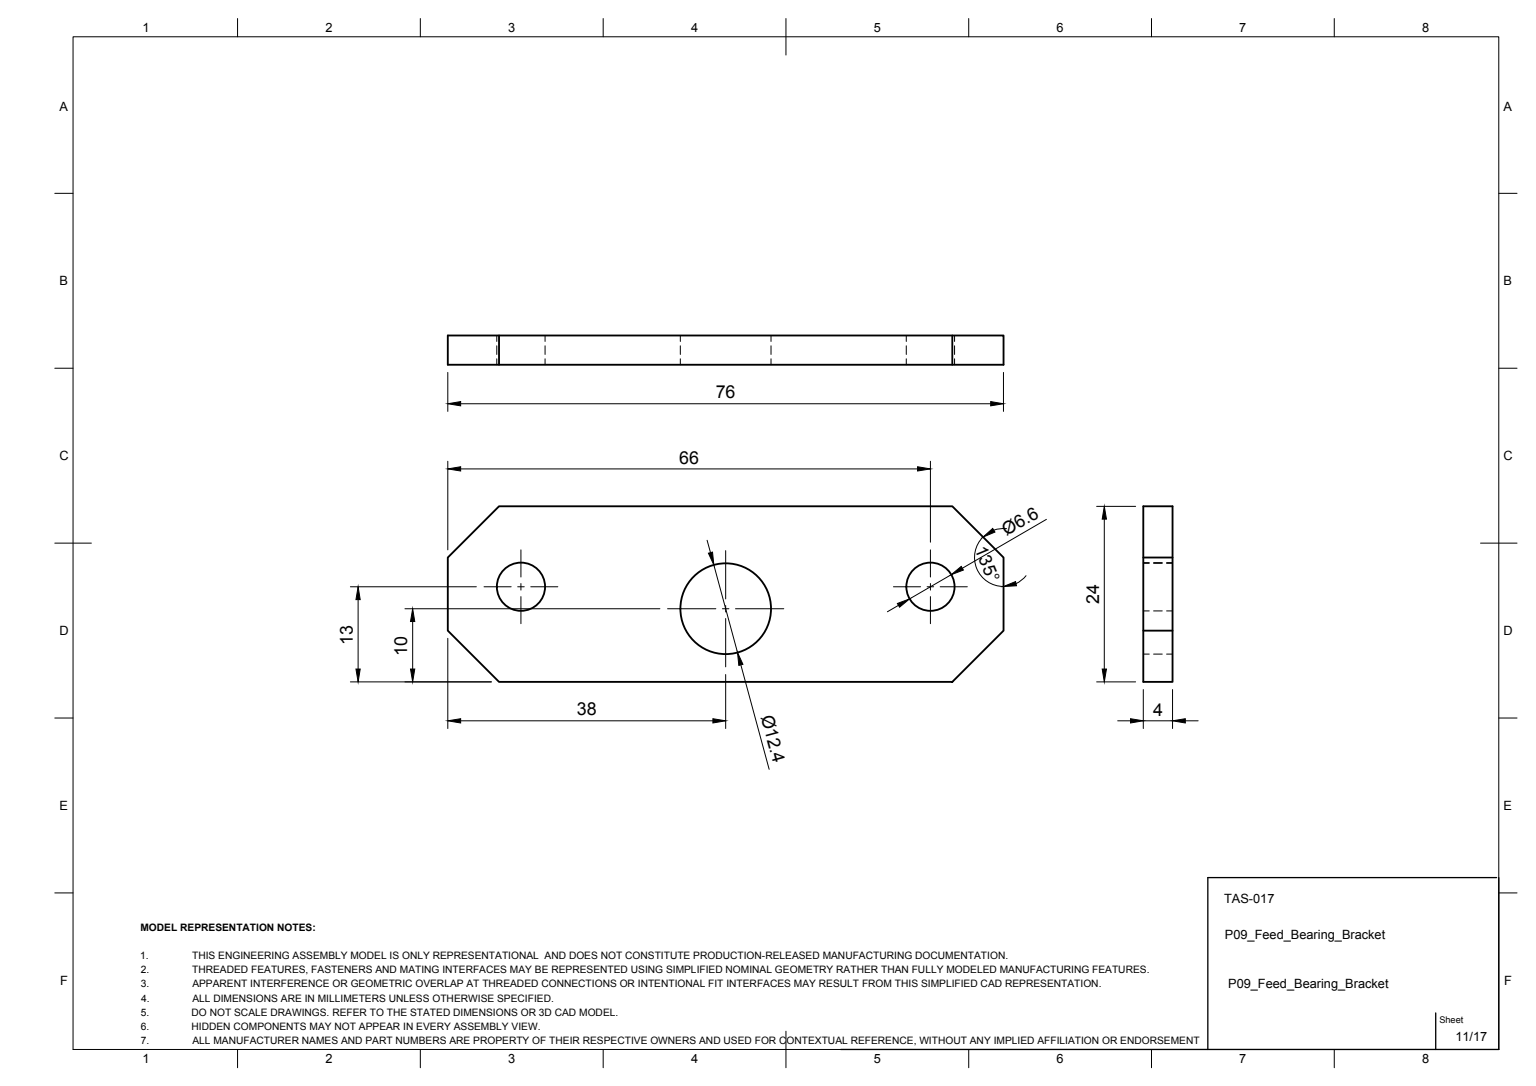
ISO-10303-21;
HEADER;
/* Generated by software containing ST-Developer
 * from STEP Tools, Inc. (www.steptools.com) 
 */

FILE_DESCRIPTION(
/* description */ ('STEP AP203'),
/* implementation_level */ '2;1');

FILE_NAME(
/* name */ 'P09_Feed_Bearing_Bracket.step',
/* time_stamp */ '2026-11-15T15:04:01-08:00',
/* author */ (''),
/* organization */ (''),
/* preprocessor_version */ 'ST-DEVELOPER v20.2',
/* originating_system */ 'Autodesk Translation Framework v15.17.0.0',
/* authorisation */ '');

FILE_SCHEMA (('AUTOMOTIVE_DESIGN { 1 0 10303 214 3 1 1 }'));
ENDSEC;

DATA;
#10=MECHANICAL_DESIGN_GEOMETRIC_PRESENTATION_REPRESENTATION('',(#297),#16598);
#219=SHAPE_REPRESENTATION_RELATIONSHIP('SRR','None',#16713,#243);
#243=ADVANCED_BREP_SHAPE_REPRESENTATION('',(#267),#16589);
#267=MANIFOLD_SOLID_BREP('Body1',#9802);
#297=STYLED_ITEM('',(#16833),#267);
#368=FACE_BOUND('',#1790,.T.);
#369=FACE_BOUND('',#1791,.T.);
#370=FACE_BOUND('',#1792,.T.);
#371=FACE_BOUND('',#1794,.T.);
#372=FACE_BOUND('',#1795,.T.);
#373=FACE_BOUND('',#1796,.T.);
#641=PLANE('',#10477);
#642=PLANE('',#10478);
#643=PLANE('',#10479);
#644=PLANE('',#10480);
#645=PLANE('',#10481);
#646=PLANE('',#10482);
#647=PLANE('',#10483);
#648=PLANE('',#10484);
#649=PLANE('',#10485);
#650=PLANE('',#10486);
#1173=FACE_OUTER_BOUND('',#1786,.T.);
#1174=FACE_OUTER_BOUND('',#1787,.T.);
#1175=FACE_OUTER_BOUND('',#1788,.T.);
#1176=FACE_OUTER_BOUND('',#1789,.T.);
#1177=FACE_OUTER_BOUND('',#1793,.T.);
#1178=FACE_OUTER_BOUND('',#1797,.T.);
#1179=FACE_OUTER_BOUND('',#1798,.T.);
#1180=FACE_OUTER_BOUND('',#1799,.T.);
#1181=FACE_OUTER_BOUND('',#1800,.T.);
#1182=FACE_OUTER_BOUND('',#1801,.T.);
#1183=FACE_OUTER_BOUND('',#1802,.T.);
#1184=FACE_OUTER_BOUND('',#1803,.T.);
#1185=FACE_OUTER_BOUND('',#1804,.T.);
#1786=EDGE_LOOP('',(#7815,#7816,#7817,#7818));
#1787=EDGE_LOOP('',(#7819,#7820,#7821,#7822));
#1788=EDGE_LOOP('',(#7823,#7824,#7825,#7826));
#1789=EDGE_LOOP('',(#7827,#7828,#7829,#7830,#7831,#7832,#7833,#7834));
#1790=EDGE_LOOP('',(#7835));
#1791=EDGE_LOOP('',(#7836));
#1792=EDGE_LOOP('',(#7837));
#1793=EDGE_LOOP('',(#7838,#7839,#7840,#7841,#7842,#7843,#7844,#7845));
#1794=EDGE_LOOP('',(#7846));
#1795=EDGE_LOOP('',(#7847));
#1796=EDGE_LOOP('',(#7848));
#1797=EDGE_LOOP('',(#7849,#7850,#7851,#7852));
#1798=EDGE_LOOP('',(#7853,#7854,#7855,#7856));
#1799=EDGE_LOOP('',(#7857,#7858,#7859,#7860));
#1800=EDGE_LOOP('',(#7861,#7862,#7863,#7864));
#1801=EDGE_LOOP('',(#7865,#7866,#7867,#7868));
#1802=EDGE_LOOP('',(#7869,#7870,#7871,#7872));
#1803=EDGE_LOOP('',(#7873,#7874,#7875,#7876));
#1804=EDGE_LOOP('',(#7877,#7878,#7879,#7880));
#2626=LINE('',#15082,#3674);
#2627=LINE('',#15088,#3675);
#2628=LINE('',#15094,#3676);
#2629=LINE('',#15099,#3677);
#2630=LINE('',#15101,#3678);
#2631=LINE('',#15103,#3679);
#2632=LINE('',#15105,#3680);
#2633=LINE('',#15107,#3681);
#2634=LINE('',#15109,#3682);
#2635=LINE('',#15111,#3683);
#2636=LINE('',#15112,#3684);
#2637=LINE('',#15116,#3685);
#2638=LINE('',#15118,#3686);
#2639=LINE('',#15120,#3687);
#2640=LINE('',#15122,#3688);
#2641=LINE('',#15124,#3689);
#2642=LINE('',#15126,#3690);
#2643=LINE('',#15128,#3691);
#2644=LINE('',#15129,#3692);
#2645=LINE('',#15131,#3693);
#2646=LINE('',#15132,#3694);
#2647=LINE('',#15134,#3695);
#2648=LINE('',#15136,#3696);
#2649=LINE('',#15138,#3697);
#2650=LINE('',#15140,#3698);
#2651=LINE('',#15142,#3699);
#2652=LINE('',#15144,#3700);
#3674=VECTOR('',#12206,3.3);
#3675=VECTOR('',#12213,3.3);
#3676=VECTOR('',#12220,6.2);
#3677=VECTOR('',#12225,1000.);
#3678=VECTOR('',#12226,1000.);
#3679=VECTOR('',#12227,1000.);
#3680=VECTOR('',#12228,1000.);
#3681=VECTOR('',#12229,1000.);
#3682=VECTOR('',#12230,1000.);
#3683=VECTOR('',#12231,1000.);
#3684=VECTOR('',#12232,1000.);
#3685=VECTOR('',#12235,1000.);
#3686=VECTOR('',#12236,1000.);
#3687=VECTOR('',#12237,1000.);
#3688=VECTOR('',#12238,1000.);
#3689=VECTOR('',#12239,1000.);
#3690=VECTOR('',#12240,1000.);
#3691=VECTOR('',#12241,1000.);
#3692=VECTOR('',#12242,1000.);
#3693=VECTOR('',#12245,1000.);
#3694=VECTOR('',#12246,1000.);
#3695=VECTOR('',#12249,1000.);
#3696=VECTOR('',#12252,1000.);
#3697=VECTOR('',#12255,1000.);
#3698=VECTOR('',#12258,1000.);
#3699=VECTOR('',#12261,1000.);
#3700=VECTOR('',#12264,1000.);
#4336=CIRCLE('',#10469,3.3);
#4337=CIRCLE('',#10470,3.3);
#4338=CIRCLE('',#10472,3.3);
#4339=CIRCLE('',#10473,3.3);
#4340=CIRCLE('',#10475,6.2);
#4341=CIRCLE('',#10476,6.2);
#4860=VERTEX_POINT('',#15079);
#4861=VERTEX_POINT('',#15081);
#4862=VERTEX_POINT('',#15085);
#4863=VERTEX_POINT('',#15087);
#4864=VERTEX_POINT('',#15091);
#4865=VERTEX_POINT('',#15093);
#4866=VERTEX_POINT('',#15097);
#4867=VERTEX_POINT('',#15098);
#4868=VERTEX_POINT('',#15100);
#4869=VERTEX_POINT('',#15102);
#4870=VERTEX_POINT('',#15104);
#4871=VERTEX_POINT('',#15106);
#4872=VERTEX_POINT('',#15108);
#4873=VERTEX_POINT('',#15110);
#4874=VERTEX_POINT('',#15114);
#4875=VERTEX_POINT('',#15115);
#4876=VERTEX_POINT('',#15117);
#4877=VERTEX_POINT('',#15119);
#4878=VERTEX_POINT('',#15121);
#4879=VERTEX_POINT('',#15123);
#4880=VERTEX_POINT('',#15125);
#4881=VERTEX_POINT('',#15127);
#5920=EDGE_CURVE('',#4860,#4860,#4336,.T.);
#5921=EDGE_CURVE('',#4860,#4861,#2626,.T.);
#5922=EDGE_CURVE('',#4861,#4861,#4337,.T.);
#5923=EDGE_CURVE('',#4862,#4862,#4338,.T.);
#5924=EDGE_CURVE('',#4862,#4863,#2627,.T.);
#5925=EDGE_CURVE('',#4863,#4863,#4339,.T.);
#5926=EDGE_CURVE('',#4864,#4864,#4340,.T.);
#5927=EDGE_CURVE('',#4864,#4865,#2628,.T.);
#5928=EDGE_CURVE('',#4865,#4865,#4341,.T.);
#5929=EDGE_CURVE('',#4866,#4867,#2629,.T.);
#5930=EDGE_CURVE('',#4867,#4868,#2630,.T.);
#5931=EDGE_CURVE('',#4868,#4869,#2631,.T.);
#5932=EDGE_CURVE('',#4869,#4870,#2632,.T.);
#5933=EDGE_CURVE('',#4870,#4871,#2633,.T.);
#5934=EDGE_CURVE('',#4871,#4872,#2634,.T.);
#5935=EDGE_CURVE('',#4872,#4873,#2635,.T.);
#5936=EDGE_CURVE('',#4873,#4866,#2636,.T.);
#5937=EDGE_CURVE('',#4874,#4875,#2637,.T.);
#5938=EDGE_CURVE('',#4876,#4874,#2638,.T.);
#5939=EDGE_CURVE('',#4877,#4876,#2639,.T.);
#5940=EDGE_CURVE('',#4878,#4877,#2640,.T.);
#5941=EDGE_CURVE('',#4879,#4878,#2641,.T.);
#5942=EDGE_CURVE('',#4880,#4879,#2642,.T.);
#5943=EDGE_CURVE('',#4881,#4880,#2643,.T.);
#5944=EDGE_CURVE('',#4875,#4881,#2644,.T.);
#5945=EDGE_CURVE('',#4867,#4875,#2645,.T.);
#5946=EDGE_CURVE('',#4866,#4874,#2646,.T.);
#5947=EDGE_CURVE('',#4868,#4881,#2647,.T.);
#5948=EDGE_CURVE('',#4869,#4880,#2648,.T.);
#5949=EDGE_CURVE('',#4870,#4879,#2649,.T.);
#5950=EDGE_CURVE('',#4871,#4878,#2650,.T.);
#5951=EDGE_CURVE('',#4872,#4877,#2651,.T.);
#5952=EDGE_CURVE('',#4873,#4876,#2652,.T.);
#7815=ORIENTED_EDGE('',*,*,#5920,.T.);
#7816=ORIENTED_EDGE('',*,*,#5921,.T.);
#7817=ORIENTED_EDGE('',*,*,#5922,.F.);
#7818=ORIENTED_EDGE('',*,*,#5921,.F.);
#7819=ORIENTED_EDGE('',*,*,#5923,.T.);
#7820=ORIENTED_EDGE('',*,*,#5924,.T.);
#7821=ORIENTED_EDGE('',*,*,#5925,.F.);
#7822=ORIENTED_EDGE('',*,*,#5924,.F.);
#7823=ORIENTED_EDGE('',*,*,#5926,.T.);
#7824=ORIENTED_EDGE('',*,*,#5927,.T.);
#7825=ORIENTED_EDGE('',*,*,#5928,.F.);
#7826=ORIENTED_EDGE('',*,*,#5927,.F.);
#7827=ORIENTED_EDGE('',*,*,#5929,.T.);
#7828=ORIENTED_EDGE('',*,*,#5930,.T.);
#7829=ORIENTED_EDGE('',*,*,#5931,.T.);
#7830=ORIENTED_EDGE('',*,*,#5932,.T.);
#7831=ORIENTED_EDGE('',*,*,#5933,.T.);
#7832=ORIENTED_EDGE('',*,*,#5934,.T.);
#7833=ORIENTED_EDGE('',*,*,#5935,.T.);
#7834=ORIENTED_EDGE('',*,*,#5936,.T.);
#7835=ORIENTED_EDGE('',*,*,#5926,.F.);
#7836=ORIENTED_EDGE('',*,*,#5920,.F.);
#7837=ORIENTED_EDGE('',*,*,#5923,.F.);
#7838=ORIENTED_EDGE('',*,*,#5937,.F.);
#7839=ORIENTED_EDGE('',*,*,#5938,.F.);
#7840=ORIENTED_EDGE('',*,*,#5939,.F.);
#7841=ORIENTED_EDGE('',*,*,#5940,.F.);
#7842=ORIENTED_EDGE('',*,*,#5941,.F.);
#7843=ORIENTED_EDGE('',*,*,#5942,.F.);
#7844=ORIENTED_EDGE('',*,*,#5943,.F.);
#7845=ORIENTED_EDGE('',*,*,#5944,.F.);
#7846=ORIENTED_EDGE('',*,*,#5928,.T.);
#7847=ORIENTED_EDGE('',*,*,#5925,.T.);
#7848=ORIENTED_EDGE('',*,*,#5922,.T.);
#7849=ORIENTED_EDGE('',*,*,#5937,.T.);
#7850=ORIENTED_EDGE('',*,*,#5945,.F.);
#7851=ORIENTED_EDGE('',*,*,#5929,.F.);
#7852=ORIENTED_EDGE('',*,*,#5946,.T.);
#7853=ORIENTED_EDGE('',*,*,#5944,.T.);
#7854=ORIENTED_EDGE('',*,*,#5947,.F.);
#7855=ORIENTED_EDGE('',*,*,#5930,.F.);
#7856=ORIENTED_EDGE('',*,*,#5945,.T.);
#7857=ORIENTED_EDGE('',*,*,#5943,.T.);
#7858=ORIENTED_EDGE('',*,*,#5948,.F.);
#7859=ORIENTED_EDGE('',*,*,#5931,.F.);
#7860=ORIENTED_EDGE('',*,*,#5947,.T.);
#7861=ORIENTED_EDGE('',*,*,#5942,.T.);
#7862=ORIENTED_EDGE('',*,*,#5949,.F.);
#7863=ORIENTED_EDGE('',*,*,#5932,.F.);
#7864=ORIENTED_EDGE('',*,*,#5948,.T.);
#7865=ORIENTED_EDGE('',*,*,#5941,.T.);
#7866=ORIENTED_EDGE('',*,*,#5950,.F.);
#7867=ORIENTED_EDGE('',*,*,#5933,.F.);
#7868=ORIENTED_EDGE('',*,*,#5949,.T.);
#7869=ORIENTED_EDGE('',*,*,#5940,.T.);
#7870=ORIENTED_EDGE('',*,*,#5951,.F.);
#7871=ORIENTED_EDGE('',*,*,#5934,.F.);
#7872=ORIENTED_EDGE('',*,*,#5950,.T.);
#7873=ORIENTED_EDGE('',*,*,#5939,.T.);
#7874=ORIENTED_EDGE('',*,*,#5952,.F.);
#7875=ORIENTED_EDGE('',*,*,#5935,.F.);
#7876=ORIENTED_EDGE('',*,*,#5951,.T.);
#7877=ORIENTED_EDGE('',*,*,#5938,.T.);
#7878=ORIENTED_EDGE('',*,*,#5946,.F.);
#7879=ORIENTED_EDGE('',*,*,#5936,.F.);
#7880=ORIENTED_EDGE('',*,*,#5952,.T.);
#9219=CYLINDRICAL_SURFACE('',#10468,3.3);
#9220=CYLINDRICAL_SURFACE('',#10471,3.3);
#9221=CYLINDRICAL_SURFACE('',#10474,6.2);
#9498=ADVANCED_FACE('',(#1173),#9219,.F.);
#9499=ADVANCED_FACE('',(#1174),#9220,.F.);
#9500=ADVANCED_FACE('',(#1175),#9221,.F.);
#9501=ADVANCED_FACE('',(#1176,#368,#369,#370),#641,.T.);
#9502=ADVANCED_FACE('',(#1177,#371,#372,#373),#642,.F.);
#9503=ADVANCED_FACE('',(#1178),#643,.F.);
#9504=ADVANCED_FACE('',(#1179),#644,.F.);
#9505=ADVANCED_FACE('',(#1180),#645,.F.);
#9506=ADVANCED_FACE('',(#1181),#646,.F.);
#9507=ADVANCED_FACE('',(#1182),#647,.F.);
#9508=ADVANCED_FACE('',(#1183),#648,.F.);
#9509=ADVANCED_FACE('',(#1184),#649,.F.);
#9510=ADVANCED_FACE('',(#1185),#650,.F.);
#9802=CLOSED_SHELL('',(#9498,#9499,#9500,#9501,#9502,#9503,#9504,#9505,
#9506,#9507,#9508,#9509,#9510));
#10467=AXIS2_PLACEMENT_3D('',#15077,#12200,#12201);
#10468=AXIS2_PLACEMENT_3D('',#15078,#12202,#12203);
#10469=AXIS2_PLACEMENT_3D('',#15080,#12204,#12205);
#10470=AXIS2_PLACEMENT_3D('',#15083,#12207,#12208);
#10471=AXIS2_PLACEMENT_3D('',#15084,#12209,#12210);
#10472=AXIS2_PLACEMENT_3D('',#15086,#12211,#12212);
#10473=AXIS2_PLACEMENT_3D('',#15089,#12214,#12215);
#10474=AXIS2_PLACEMENT_3D('',#15090,#12216,#12217);
#10475=AXIS2_PLACEMENT_3D('',#15092,#12218,#12219);
#10476=AXIS2_PLACEMENT_3D('',#15095,#12221,#12222);
#10477=AXIS2_PLACEMENT_3D('',#15096,#12223,#12224);
#10478=AXIS2_PLACEMENT_3D('',#15113,#12233,#12234);
#10479=AXIS2_PLACEMENT_3D('',#15130,#12243,#12244);
#10480=AXIS2_PLACEMENT_3D('',#15133,#12247,#12248);
#10481=AXIS2_PLACEMENT_3D('',#15135,#12250,#12251);
#10482=AXIS2_PLACEMENT_3D('',#15137,#12253,#12254);
#10483=AXIS2_PLACEMENT_3D('',#15139,#12256,#12257);
#10484=AXIS2_PLACEMENT_3D('',#15141,#12259,#12260);
#10485=AXIS2_PLACEMENT_3D('',#15143,#12262,#12263);
#10486=AXIS2_PLACEMENT_3D('',#15145,#12265,#12266);
#12200=DIRECTION('axis',(0.,0.,1.));
#12201=DIRECTION('refdir',(1.,0.,0.));
#12202=DIRECTION('center_axis',(0.,0.,-1.));
#12203=DIRECTION('ref_axis',(-1.,0.,0.));
#12204=DIRECTION('center_axis',(0.,0.,1.));
#12205=DIRECTION('ref_axis',(1.,0.,0.));
#12206=DIRECTION('',(0.,0.,-1.));
#12207=DIRECTION('center_axis',(0.,0.,1.));
#12208=DIRECTION('ref_axis',(1.,0.,0.));
#12209=DIRECTION('center_axis',(0.,0.,-1.));
#12210=DIRECTION('ref_axis',(-1.,0.,0.));
#12211=DIRECTION('center_axis',(0.,0.,1.));
#12212=DIRECTION('ref_axis',(1.,0.,0.));
#12213=DIRECTION('',(0.,0.,-1.));
#12214=DIRECTION('center_axis',(0.,0.,1.));
#12215=DIRECTION('ref_axis',(1.,0.,0.));
#12216=DIRECTION('center_axis',(0.,0.,-1.));
#12217=DIRECTION('ref_axis',(-1.,0.,0.));
#12218=DIRECTION('center_axis',(0.,0.,1.));
#12219=DIRECTION('ref_axis',(1.,0.,0.));
#12220=DIRECTION('',(0.,0.,-1.));
#12221=DIRECTION('center_axis',(0.,0.,1.));
#12222=DIRECTION('ref_axis',(1.,0.,0.));
#12223=DIRECTION('center_axis',(0.,0.,1.));
#12224=DIRECTION('ref_axis',(1.,0.,0.));
#12225=DIRECTION('',(0.,-1.,0.));
#12226=DIRECTION('',(0.707106781186548,-0.707106781186548,0.));
#12227=DIRECTION('',(1.,0.,0.));
#12228=DIRECTION('',(0.707106781186548,0.707106781186548,0.));
#12229=DIRECTION('',(0.,1.,0.));
#12230=DIRECTION('',(-0.707106781186548,0.707106781186548,0.));
#12231=DIRECTION('',(-1.,0.,0.));
#12232=DIRECTION('',(-0.707106781186548,-0.707106781186548,0.));
#12233=DIRECTION('center_axis',(0.,0.,1.));
#12234=DIRECTION('ref_axis',(1.,0.,0.));
#12235=DIRECTION('',(0.,-1.,0.));
#12236=DIRECTION('',(-0.707106781186548,-0.707106781186548,0.));
#12237=DIRECTION('',(-1.,0.,0.));
#12238=DIRECTION('',(-0.707106781186548,0.707106781186548,0.));
#12239=DIRECTION('',(0.,1.,0.));
#12240=DIRECTION('',(0.707106781186548,0.707106781186548,0.));
#12241=DIRECTION('',(1.,0.,0.));
#12242=DIRECTION('',(0.707106781186548,-0.707106781186548,0.));
#12243=DIRECTION('center_axis',(1.,0.,0.));
#12244=DIRECTION('ref_axis',(0.,0.,-1.));
#12245=DIRECTION('',(0.,0.,-1.));
#12246=DIRECTION('',(0.,0.,-1.));
#12247=DIRECTION('center_axis',(0.707106781186548,0.707106781186547,0.));
#12248=DIRECTION('ref_axis',(-0.707106781186547,0.707106781186548,0.));
#12249=DIRECTION('',(0.,0.,-1.));
#12250=DIRECTION('center_axis',(0.,1.,0.));
#12251=DIRECTION('ref_axis',(0.,0.,1.));
#12252=DIRECTION('',(0.,0.,-1.));
#12253=DIRECTION('center_axis',(-0.707106781186548,0.707106781186547,0.));
#12254=DIRECTION('ref_axis',(-0.707106781186547,-0.707106781186548,0.));
#12255=DIRECTION('',(0.,0.,-1.));
#12256=DIRECTION('center_axis',(-1.,0.,0.));
#12257=DIRECTION('ref_axis',(0.,0.,1.));
#12258=DIRECTION('',(0.,0.,-1.));
#12259=DIRECTION('center_axis',(-0.707106781186548,-0.707106781186547,0.));
#12260=DIRECTION('ref_axis',(0.707106781186547,-0.707106781186548,0.));
#12261=DIRECTION('',(0.,0.,-1.));
#12262=DIRECTION('center_axis',(0.,-1.,0.));
#12263=DIRECTION('ref_axis',(0.,0.,-1.));
#12264=DIRECTION('',(0.,0.,-1.));
#12265=DIRECTION('center_axis',(0.707106781186548,-0.707106781186547,0.));
#12266=DIRECTION('ref_axis',(0.707106781186547,0.707106781186548,0.));
#15077=CARTESIAN_POINT('',(0.,0.,0.));
#15078=CARTESIAN_POINT('Origin',(28.,3.,4.));
#15079=CARTESIAN_POINT('',(31.3,3.,4.));
#15080=CARTESIAN_POINT('Origin',(28.,3.,4.));
#15081=CARTESIAN_POINT('',(31.3,3.,0.));
#15082=CARTESIAN_POINT('',(31.3,3.,4.));
#15083=CARTESIAN_POINT('Origin',(28.,3.,0.));
#15084=CARTESIAN_POINT('Origin',(-28.,3.,4.));
#15085=CARTESIAN_POINT('',(-24.7,3.,4.));
#15086=CARTESIAN_POINT('Origin',(-28.,3.,4.));
#15087=CARTESIAN_POINT('',(-24.7,3.,0.));
#15088=CARTESIAN_POINT('',(-24.7,3.,4.));
#15089=CARTESIAN_POINT('Origin',(-28.,3.,0.));
#15090=CARTESIAN_POINT('Origin',(0.,0.,4.));
#15091=CARTESIAN_POINT('',(6.2,-7.59281015471359E-16,4.));
#15092=CARTESIAN_POINT('Origin',(0.,0.,4.));
#15093=CARTESIAN_POINT('',(6.2,-7.59281015471359E-16,5.55111512312578E-16));
#15094=CARTESIAN_POINT('',(6.2,-7.59281015471359E-16,4.));
#15095=CARTESIAN_POINT('Origin',(0.,0.,0.));
#15096=CARTESIAN_POINT('Origin',(0.,0.,4.));
#15097=CARTESIAN_POINT('',(-38.,7.,4.));
#15098=CARTESIAN_POINT('',(-38.,-3.,4.));
#15099=CARTESIAN_POINT('',(-38.,7.,4.));
#15100=CARTESIAN_POINT('',(-31.,-10.,4.));
#15101=CARTESIAN_POINT('',(-38.,-3.,4.));
#15102=CARTESIAN_POINT('',(31.,-10.,4.));
#15103=CARTESIAN_POINT('',(-31.,-10.,4.));
#15104=CARTESIAN_POINT('',(38.,-3.,4.));
#15105=CARTESIAN_POINT('',(31.,-10.,4.));
#15106=CARTESIAN_POINT('',(38.,7.,4.));
#15107=CARTESIAN_POINT('',(38.,-3.,4.));
#15108=CARTESIAN_POINT('',(31.,14.,4.));
#15109=CARTESIAN_POINT('',(38.,7.,4.));
#15110=CARTESIAN_POINT('',(-31.,14.,4.));
#15111=CARTESIAN_POINT('',(31.,14.,4.));
#15112=CARTESIAN_POINT('',(-31.,14.,4.));
#15113=CARTESIAN_POINT('Origin',(0.,0.,0.));
#15114=CARTESIAN_POINT('',(-38.,7.,0.));
#15115=CARTESIAN_POINT('',(-38.,-3.,0.));
#15116=CARTESIAN_POINT('',(-38.,7.,0.));
#15117=CARTESIAN_POINT('',(-31.,14.,0.));
#15118=CARTESIAN_POINT('',(-31.,14.,0.));
#15119=CARTESIAN_POINT('',(31.,14.,0.));
#15120=CARTESIAN_POINT('',(31.,14.,0.));
#15121=CARTESIAN_POINT('',(38.,7.,0.));
#15122=CARTESIAN_POINT('',(38.,7.,0.));
#15123=CARTESIAN_POINT('',(38.,-3.,0.));
#15124=CARTESIAN_POINT('',(38.,-3.,0.));
#15125=CARTESIAN_POINT('',(31.,-10.,0.));
#15126=CARTESIAN_POINT('',(31.,-10.,0.));
#15127=CARTESIAN_POINT('',(-31.,-10.,0.));
#15128=CARTESIAN_POINT('',(-31.,-10.,0.));
#15129=CARTESIAN_POINT('',(-38.,-3.,0.));
#15130=CARTESIAN_POINT('Origin',(-38.,7.,4.));
#15131=CARTESIAN_POINT('',(-38.,-3.,4.));
#15132=CARTESIAN_POINT('',(-38.,7.,4.));
#15133=CARTESIAN_POINT('Origin',(-38.,-3.,4.));
#15134=CARTESIAN_POINT('',(-31.,-10.,4.));
#15135=CARTESIAN_POINT('Origin',(-31.,-10.,4.));
#15136=CARTESIAN_POINT('',(31.,-10.,4.));
#15137=CARTESIAN_POINT('Origin',(31.,-10.,4.));
#15138=CARTESIAN_POINT('',(38.,-3.,4.));
#15139=CARTESIAN_POINT('Origin',(38.,-3.,4.));
#15140=CARTESIAN_POINT('',(38.,7.,4.));
#15141=CARTESIAN_POINT('Origin',(38.,7.,4.));
#15142=CARTESIAN_POINT('',(31.,14.,4.));
#15143=CARTESIAN_POINT('Origin',(31.,14.,4.));
#15144=CARTESIAN_POINT('',(-31.,14.,4.));
#15145=CARTESIAN_POINT('Origin',(-31.,14.,4.));
#16563=UNCERTAINTY_MEASURE_WITH_UNIT(LENGTH_MEASURE(0.01),#16599,
'DISTANCE_ACCURACY_VALUE',
'Maximum model space distance between geometric entities at asserted c
onnectivities');
#16572=UNCERTAINTY_MEASURE_WITH_UNIT(LENGTH_MEASURE(0.01),#16599,
'DISTANCE_ACCURACY_VALUE',
'Maximum model space distance between geometric entities at asserted c
onnectivities');
#16589=(
GEOMETRIC_REPRESENTATION_CONTEXT(3)
GLOBAL_UNCERTAINTY_ASSIGNED_CONTEXT((#16563))
GLOBAL_UNIT_ASSIGNED_CONTEXT((#16599,#16601,#16602))
REPRESENTATION_CONTEXT('','3D')
);
#16598=(
GEOMETRIC_REPRESENTATION_CONTEXT(3)
GLOBAL_UNCERTAINTY_ASSIGNED_CONTEXT((#16572))
GLOBAL_UNIT_ASSIGNED_CONTEXT((#16599,#16601,#16602))
REPRESENTATION_CONTEXT('','3D')
);
#16599=(
LENGTH_UNIT()
NAMED_UNIT(*)
SI_UNIT(.MILLI.,.METRE.)
);
#16601=(
NAMED_UNIT(*)
PLANE_ANGLE_UNIT()
SI_UNIT($,.RADIAN.)
);
#16602=(
NAMED_UNIT(*)
SI_UNIT($,.STERADIAN.)
SOLID_ANGLE_UNIT()
);
#16619=SHAPE_DEFINITION_REPRESENTATION(#16644,#16713);
#16644=PRODUCT_DEFINITION_SHAPE('',$,#16739);
#16713=SHAPE_REPRESENTATION('',(#10467),#16589);
#16722=PRODUCT_DEFINITION_CONTEXT('part definition',#16799,'design');
#16739=PRODUCT_DEFINITION('P09_Feed_Bearing_Bracket',
'P09_Feed_Bearing_Bracket',#16764,#16722);
#16764=PRODUCT_DEFINITION_FORMATION('',$,#16817);
#16799=APPLICATION_CONTEXT(
'Core Data for Automotive Mechanical Design Process');
#16800=PRODUCT_CONTEXT('part definition',#16799,'mechanical');
#16817=PRODUCT('P09_Feed_Bearing_Bracket','P09_Feed_Bearing_Bracket',$,
(#16800));
#16833=PRESENTATION_STYLE_ASSIGNMENT((#16842));
#16842=SURFACE_STYLE_USAGE(.BOTH.,#16851);
#16851=SURFACE_SIDE_STYLE('',(#16860));
#16860=SURFACE_STYLE_FILL_AREA(#16869);
#16869=FILL_AREA_STYLE('Blue',(#16878));
#16878=FILL_AREA_STYLE_COLOUR('Blue',#16887);
#16887=COLOUR_RGB('Blue',0.,0.4,0.8);
ENDSEC;
END-ISO-10303-21;
